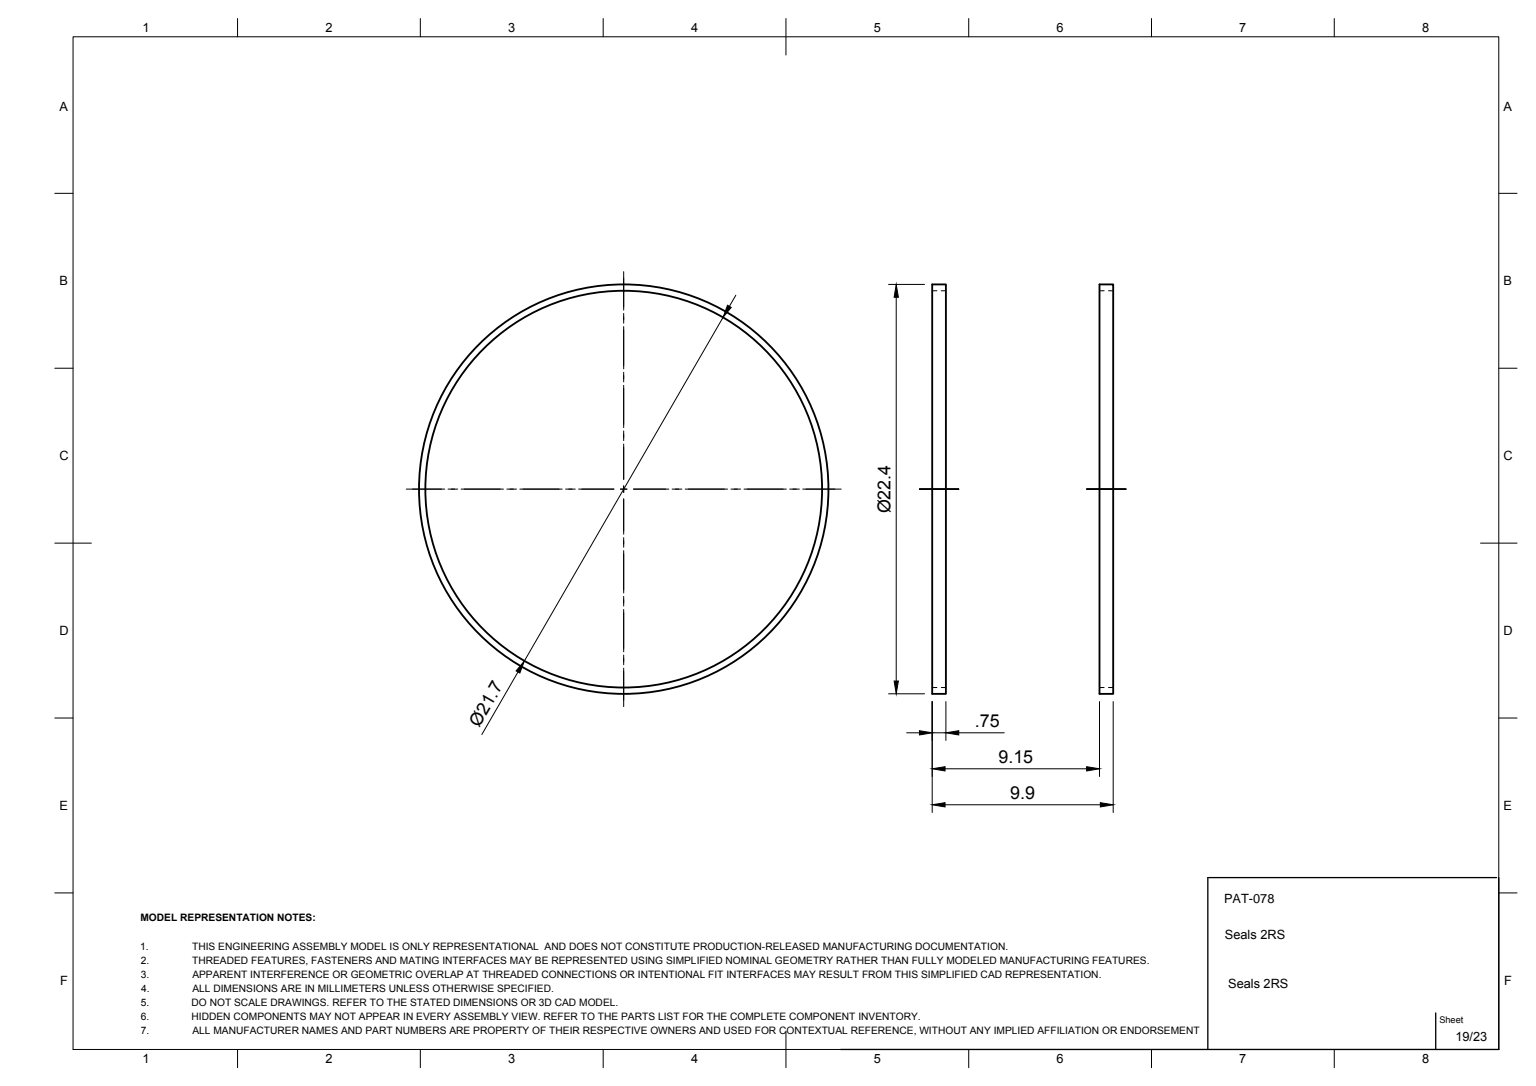
ISO-10303-21;
HEADER;
/* Generated by software containing ST-Developer
 * from STEP Tools, Inc. (www.steptools.com) 
 */

FILE_DESCRIPTION(
/* description */ ('Pedal-braked fixed caster'),
/* implementation_level */ '2;1');

FILE_NAME(
/* name */ 'Seals 2RS.step',
/* time_stamp */ '2026-10-28T03:26:52-07:00',
/* author */ (''),
/* organization */ (''),
/* preprocessor_version */ 'ST-DEVELOPER v20.2',
/* originating_system */ 'Autodesk Translation Framework v15.17.0.0',
/* authorisation */ '');

FILE_SCHEMA (('AUTOMOTIVE_DESIGN { 1 0 10303 214 3 1 1 }'));
ENDSEC;

DATA;
#10=MECHANICAL_DESIGN_GEOMETRIC_PRESENTATION_REPRESENTATION('',(#225,#226),#5734);
#185=SHAPE_REPRESENTATION_RELATIONSHIP('SRR','None',#5825,#202);
#202=ADVANCED_BREP_SHAPE_REPRESENTATION('',(#248,#249),#5729);
#225=STYLED_ITEM('',(#5984),#248);
#226=STYLED_ITEM('',(#5984),#249);
#248=MANIFOLD_SOLID_BREP('Body1',#3007);
#249=MANIFOLD_SOLID_BREP('Body2',#3008);
#286=CYLINDRICAL_SURFACE('',#3497,1.119765);
#287=CYLINDRICAL_SURFACE('',#3501,1.085235);
#288=CYLINDRICAL_SURFACE('',#3505,1.119765);
#289=CYLINDRICAL_SURFACE('',#3509,1.085235);
#332=FACE_BOUND('',#840,.T.);
#333=FACE_BOUND('',#843,.T.);
#334=FACE_BOUND('',#846,.T.);
#335=FACE_BOUND('',#849,.T.);
#458=CIRCLE('',#3495,1.119765);
#459=CIRCLE('',#3496,1.085235);
#460=CIRCLE('',#3498,1.119765);
#461=CIRCLE('',#3500,1.085235);
#462=CIRCLE('',#3503,1.119765);
#463=CIRCLE('',#3504,1.085235);
#464=CIRCLE('',#3506,1.119765);
#465=CIRCLE('',#3508,1.085235);
#624=FACE_OUTER_BOUND('',#839,.T.);
#625=FACE_OUTER_BOUND('',#841,.T.);
#626=FACE_OUTER_BOUND('',#842,.T.);
#627=FACE_OUTER_BOUND('',#844,.T.);
#628=FACE_OUTER_BOUND('',#845,.T.);
#629=FACE_OUTER_BOUND('',#847,.T.);
#630=FACE_OUTER_BOUND('',#848,.T.);
#631=FACE_OUTER_BOUND('',#850,.T.);
#839=EDGE_LOOP('',(#2580));
#840=EDGE_LOOP('',(#2581));
#841=EDGE_LOOP('',(#2582,#2583,#2584,#2585));
#842=EDGE_LOOP('',(#2586));
#843=EDGE_LOOP('',(#2587));
#844=EDGE_LOOP('',(#2588,#2589,#2590,#2591));
#845=EDGE_LOOP('',(#2592));
#846=EDGE_LOOP('',(#2593));
#847=EDGE_LOOP('',(#2594,#2595,#2596,#2597));
#848=EDGE_LOOP('',(#2598));
#849=EDGE_LOOP('',(#2599));
#850=EDGE_LOOP('',(#2600,#2601,#2602,#2603));
#1047=LINE('',#5548,#1259);
#1048=LINE('',#5553,#1260);
#1049=LINE('',#5562,#1261);
#1050=LINE('',#5567,#1262);
#1259=VECTOR('',#4329,1.119765);
#1260=VECTOR('',#4336,1.085235);
#1261=VECTOR('',#4347,1.119765);
#1262=VECTOR('',#4354,1.085235);
#1520=VERTEX_POINT('',#5541);
#1521=VERTEX_POINT('',#5543);
#1522=VERTEX_POINT('',#5546);
#1523=VERTEX_POINT('',#5550);
#1524=VERTEX_POINT('',#5555);
#1525=VERTEX_POINT('',#5557);
#1526=VERTEX_POINT('',#5560);
#1527=VERTEX_POINT('',#5564);
#1880=EDGE_CURVE('',#1520,#1520,#458,.T.);
#1881=EDGE_CURVE('',#1521,#1521,#459,.T.);
#1882=EDGE_CURVE('',#1522,#1522,#460,.T.);
#1883=EDGE_CURVE('',#1522,#1520,#1047,.T.);
#1884=EDGE_CURVE('',#1523,#1523,#461,.T.);
#1885=EDGE_CURVE('',#1523,#1521,#1048,.T.);
#1886=EDGE_CURVE('',#1524,#1524,#462,.T.);
#1887=EDGE_CURVE('',#1525,#1525,#463,.T.);
#1888=EDGE_CURVE('',#1526,#1526,#464,.T.);
#1889=EDGE_CURVE('',#1526,#1524,#1049,.T.);
#1890=EDGE_CURVE('',#1527,#1527,#465,.T.);
#1891=EDGE_CURVE('',#1527,#1525,#1050,.T.);
#2580=ORIENTED_EDGE('',*,*,#1880,.F.);
#2581=ORIENTED_EDGE('',*,*,#1881,.T.);
#2582=ORIENTED_EDGE('',*,*,#1882,.F.);
#2583=ORIENTED_EDGE('',*,*,#1883,.T.);
#2584=ORIENTED_EDGE('',*,*,#1880,.T.);
#2585=ORIENTED_EDGE('',*,*,#1883,.F.);
#2586=ORIENTED_EDGE('',*,*,#1882,.T.);
#2587=ORIENTED_EDGE('',*,*,#1884,.F.);
#2588=ORIENTED_EDGE('',*,*,#1884,.T.);
#2589=ORIENTED_EDGE('',*,*,#1885,.T.);
#2590=ORIENTED_EDGE('',*,*,#1881,.F.);
#2591=ORIENTED_EDGE('',*,*,#1885,.F.);
#2592=ORIENTED_EDGE('',*,*,#1886,.F.);
#2593=ORIENTED_EDGE('',*,*,#1887,.T.);
#2594=ORIENTED_EDGE('',*,*,#1888,.F.);
#2595=ORIENTED_EDGE('',*,*,#1889,.T.);
#2596=ORIENTED_EDGE('',*,*,#1886,.T.);
#2597=ORIENTED_EDGE('',*,*,#1889,.F.);
#2598=ORIENTED_EDGE('',*,*,#1888,.T.);
#2599=ORIENTED_EDGE('',*,*,#1890,.F.);
#2600=ORIENTED_EDGE('',*,*,#1890,.T.);
#2601=ORIENTED_EDGE('',*,*,#1891,.T.);
#2602=ORIENTED_EDGE('',*,*,#1887,.F.);
#2603=ORIENTED_EDGE('',*,*,#1891,.F.);
#2788=PLANE('',#3494);
#2789=PLANE('',#3499);
#2790=PLANE('',#3502);
#2791=PLANE('',#3507);
#2957=ADVANCED_FACE('',(#624,#332),#2788,.T.);
#2958=ADVANCED_FACE('',(#625),#286,.T.);
#2959=ADVANCED_FACE('',(#626,#333),#2789,.T.);
#2960=ADVANCED_FACE('',(#627),#287,.F.);
#2961=ADVANCED_FACE('',(#628,#334),#2790,.T.);
#2962=ADVANCED_FACE('',(#629),#288,.T.);
#2963=ADVANCED_FACE('',(#630,#335),#2791,.T.);
#2964=ADVANCED_FACE('',(#631),#289,.F.);
#3007=CLOSED_SHELL('',(#2957,#2958,#2959,#2960));
#3008=CLOSED_SHELL('',(#2961,#2962,#2963,#2964));
#3493=AXIS2_PLACEMENT_3D('',#5539,#4317,#4318);
#3494=AXIS2_PLACEMENT_3D('',#5540,#4319,#4320);
#3495=AXIS2_PLACEMENT_3D('',#5542,#4321,#4322);
#3496=AXIS2_PLACEMENT_3D('',#5544,#4323,#4324);
#3497=AXIS2_PLACEMENT_3D('',#5545,#4325,#4326);
#3498=AXIS2_PLACEMENT_3D('',#5547,#4327,#4328);
#3499=AXIS2_PLACEMENT_3D('',#5549,#4330,#4331);
#3500=AXIS2_PLACEMENT_3D('',#5551,#4332,#4333);
#3501=AXIS2_PLACEMENT_3D('',#5552,#4334,#4335);
#3502=AXIS2_PLACEMENT_3D('',#5554,#4337,#4338);
#3503=AXIS2_PLACEMENT_3D('',#5556,#4339,#4340);
#3504=AXIS2_PLACEMENT_3D('',#5558,#4341,#4342);
#3505=AXIS2_PLACEMENT_3D('',#5559,#4343,#4344);
#3506=AXIS2_PLACEMENT_3D('',#5561,#4345,#4346);
#3507=AXIS2_PLACEMENT_3D('',#5563,#4348,#4349);
#3508=AXIS2_PLACEMENT_3D('',#5565,#4350,#4351);
#3509=AXIS2_PLACEMENT_3D('',#5566,#4352,#4353);
#4317=DIRECTION('axis',(0.,0.,1.));
#4318=DIRECTION('refdir',(1.,0.,0.));
#4319=DIRECTION('center_axis',(0.,1.,0.));
#4320=DIRECTION('ref_axis',(0.,0.,1.));
#4321=DIRECTION('center_axis',(0.,-1.,0.));
#4322=DIRECTION('ref_axis',(1.,0.,0.));
#4323=DIRECTION('center_axis',(0.,-1.,0.));
#4324=DIRECTION('ref_axis',(1.,0.,0.));
#4325=DIRECTION('center_axis',(0.,-1.,0.));
#4326=DIRECTION('ref_axis',(1.,0.,0.));
#4327=DIRECTION('center_axis',(0.,-1.,0.));
#4328=DIRECTION('ref_axis',(1.,0.,0.));
#4329=DIRECTION('',(0.,1.,0.));
#4330=DIRECTION('center_axis',(0.,-1.,0.));
#4331=DIRECTION('ref_axis',(0.,0.,-1.));
#4332=DIRECTION('center_axis',(0.,-1.,0.));
#4333=DIRECTION('ref_axis',(1.,0.,0.));
#4334=DIRECTION('center_axis',(0.,-1.,0.));
#4335=DIRECTION('ref_axis',(1.,0.,0.));
#4336=DIRECTION('',(0.,1.,0.));
#4337=DIRECTION('center_axis',(0.,1.,0.));
#4338=DIRECTION('ref_axis',(0.,0.,1.));
#4339=DIRECTION('center_axis',(0.,-1.,0.));
#4340=DIRECTION('ref_axis',(1.,0.,0.));
#4341=DIRECTION('center_axis',(0.,-1.,0.));
#4342=DIRECTION('ref_axis',(1.,0.,0.));
#4343=DIRECTION('center_axis',(0.,-1.,0.));
#4344=DIRECTION('ref_axis',(1.,0.,0.));
#4345=DIRECTION('center_axis',(0.,-1.,0.));
#4346=DIRECTION('ref_axis',(1.,0.,0.));
#4347=DIRECTION('',(0.,1.,0.));
#4348=DIRECTION('center_axis',(0.,-1.,0.));
#4349=DIRECTION('ref_axis',(0.,0.,-1.));
#4350=DIRECTION('center_axis',(0.,-1.,0.));
#4351=DIRECTION('ref_axis',(1.,0.,0.));
#4352=DIRECTION('center_axis',(0.,-1.,0.));
#4353=DIRECTION('ref_axis',(1.,0.,0.));
#4354=DIRECTION('',(0.,1.,0.));
#5539=CARTESIAN_POINT('',(0.,0.,0.));
#5540=CARTESIAN_POINT('Origin',(1.119765,0.495,0.));
#5541=CARTESIAN_POINT('',(-1.119765,0.495,-1.37131662304724E-16));
#5542=CARTESIAN_POINT('Origin',(0.,0.495,0.));
#5543=CARTESIAN_POINT('',(-1.085235,0.495,-1.32902956907268E-16));
#5544=CARTESIAN_POINT('Origin',(0.,0.495,0.));
#5545=CARTESIAN_POINT('Origin',(0.,0.4575,0.));
#5546=CARTESIAN_POINT('',(-1.119765,0.42,-1.37131662304724E-16));
#5547=CARTESIAN_POINT('Origin',(0.,0.42,0.));
#5548=CARTESIAN_POINT('',(-1.119765,0.4575,-1.37131662304724E-16));
#5549=CARTESIAN_POINT('Origin',(1.085235,0.42,0.));
#5550=CARTESIAN_POINT('',(-1.085235,0.42,-1.32902956907268E-16));
#5551=CARTESIAN_POINT('Origin',(0.,0.42,0.));
#5552=CARTESIAN_POINT('Origin',(0.,0.4575,0.));
#5553=CARTESIAN_POINT('',(-1.085235,0.4575,-1.32902956907268E-16));
#5554=CARTESIAN_POINT('Origin',(1.119765,-0.42,0.));
#5555=CARTESIAN_POINT('',(-1.119765,-0.42,-1.37131662304724E-16));
#5556=CARTESIAN_POINT('Origin',(0.,-0.42,0.));
#5557=CARTESIAN_POINT('',(-1.085235,-0.42,-1.32902956907268E-16));
#5558=CARTESIAN_POINT('Origin',(0.,-0.42,0.));
#5559=CARTESIAN_POINT('Origin',(0.,-0.4575,0.));
#5560=CARTESIAN_POINT('',(-1.119765,-0.495,-1.37131662304724E-16));
#5561=CARTESIAN_POINT('Origin',(0.,-0.495,0.));
#5562=CARTESIAN_POINT('',(-1.119765,-0.4575,-1.37131662304724E-16));
#5563=CARTESIAN_POINT('Origin',(1.085235,-0.495,0.));
#5564=CARTESIAN_POINT('',(-1.085235,-0.495,-1.32902956907268E-16));
#5565=CARTESIAN_POINT('Origin',(0.,-0.495,0.));
#5566=CARTESIAN_POINT('Origin',(0.,-0.4575,0.));
#5567=CARTESIAN_POINT('',(-1.085235,-0.4575,-1.32902956907268E-16));
#5706=UNCERTAINTY_MEASURE_WITH_UNIT(LENGTH_MEASURE(0.001),#5735,
'DISTANCE_ACCURACY_VALUE',
'Maximum model space distance between geometric entities at asserted c
onnectivities');
#5711=UNCERTAINTY_MEASURE_WITH_UNIT(LENGTH_MEASURE(0.001),#5735,
'DISTANCE_ACCURACY_VALUE',
'Maximum model space distance between geometric entities at asserted c
onnectivities');
#5729=(
GEOMETRIC_REPRESENTATION_CONTEXT(3)
GLOBAL_UNCERTAINTY_ASSIGNED_CONTEXT((#5706))
GLOBAL_UNIT_ASSIGNED_CONTEXT((#5735,#5737,#5738))
REPRESENTATION_CONTEXT('','3D')
);
#5734=(
GEOMETRIC_REPRESENTATION_CONTEXT(3)
GLOBAL_UNCERTAINTY_ASSIGNED_CONTEXT((#5711))
GLOBAL_UNIT_ASSIGNED_CONTEXT((#5735,#5737,#5738))
REPRESENTATION_CONTEXT('','3D')
);
#5735=(
LENGTH_UNIT()
NAMED_UNIT(*)
SI_UNIT(.CENTI.,.METRE.)
);
#5737=(
NAMED_UNIT(*)
PLANE_ANGLE_UNIT()
SI_UNIT($,.RADIAN.)
);
#5738=(
NAMED_UNIT(*)
SI_UNIT($,.STERADIAN.)
SOLID_ANGLE_UNIT()
);
#5756=SHAPE_DEFINITION_REPRESENTATION(#5788,#5825);
#5788=PRODUCT_DEFINITION_SHAPE('',$,#5848);
#5825=SHAPE_REPRESENTATION('',(#3493),#5729);
#5830=PRODUCT_DEFINITION_CONTEXT('part definition',#5898,'design');
#5848=PRODUCT_DEFINITION('Seals 2RS','Seals 2RS',#5870,#5830);
#5870=PRODUCT_DEFINITION_FORMATION('',$,#5917);
#5898=APPLICATION_CONTEXT(
'Core Data for Automotive Mechanical Design Process');
#5899=PRODUCT_CONTEXT('part definition',#5898,'mechanical');
#5917=PRODUCT('Seals 2RS','Seals 2RS','Seals 2RS',(#5899));
#5978=COLOUR_RGB('Grey',0.48,0.52,0.57);
#5979=FILL_AREA_STYLE_COLOUR('',#5978);
#5980=FILL_AREA_STYLE('',(#5979));
#5981=SURFACE_STYLE_FILL_AREA(#5980);
#5982=SURFACE_SIDE_STYLE('',(#5981));
#5983=SURFACE_STYLE_USAGE(.BOTH.,#5982);
#5984=PRESENTATION_STYLE_ASSIGNMENT((#5983));
ENDSEC;
END-ISO-10303-21;
